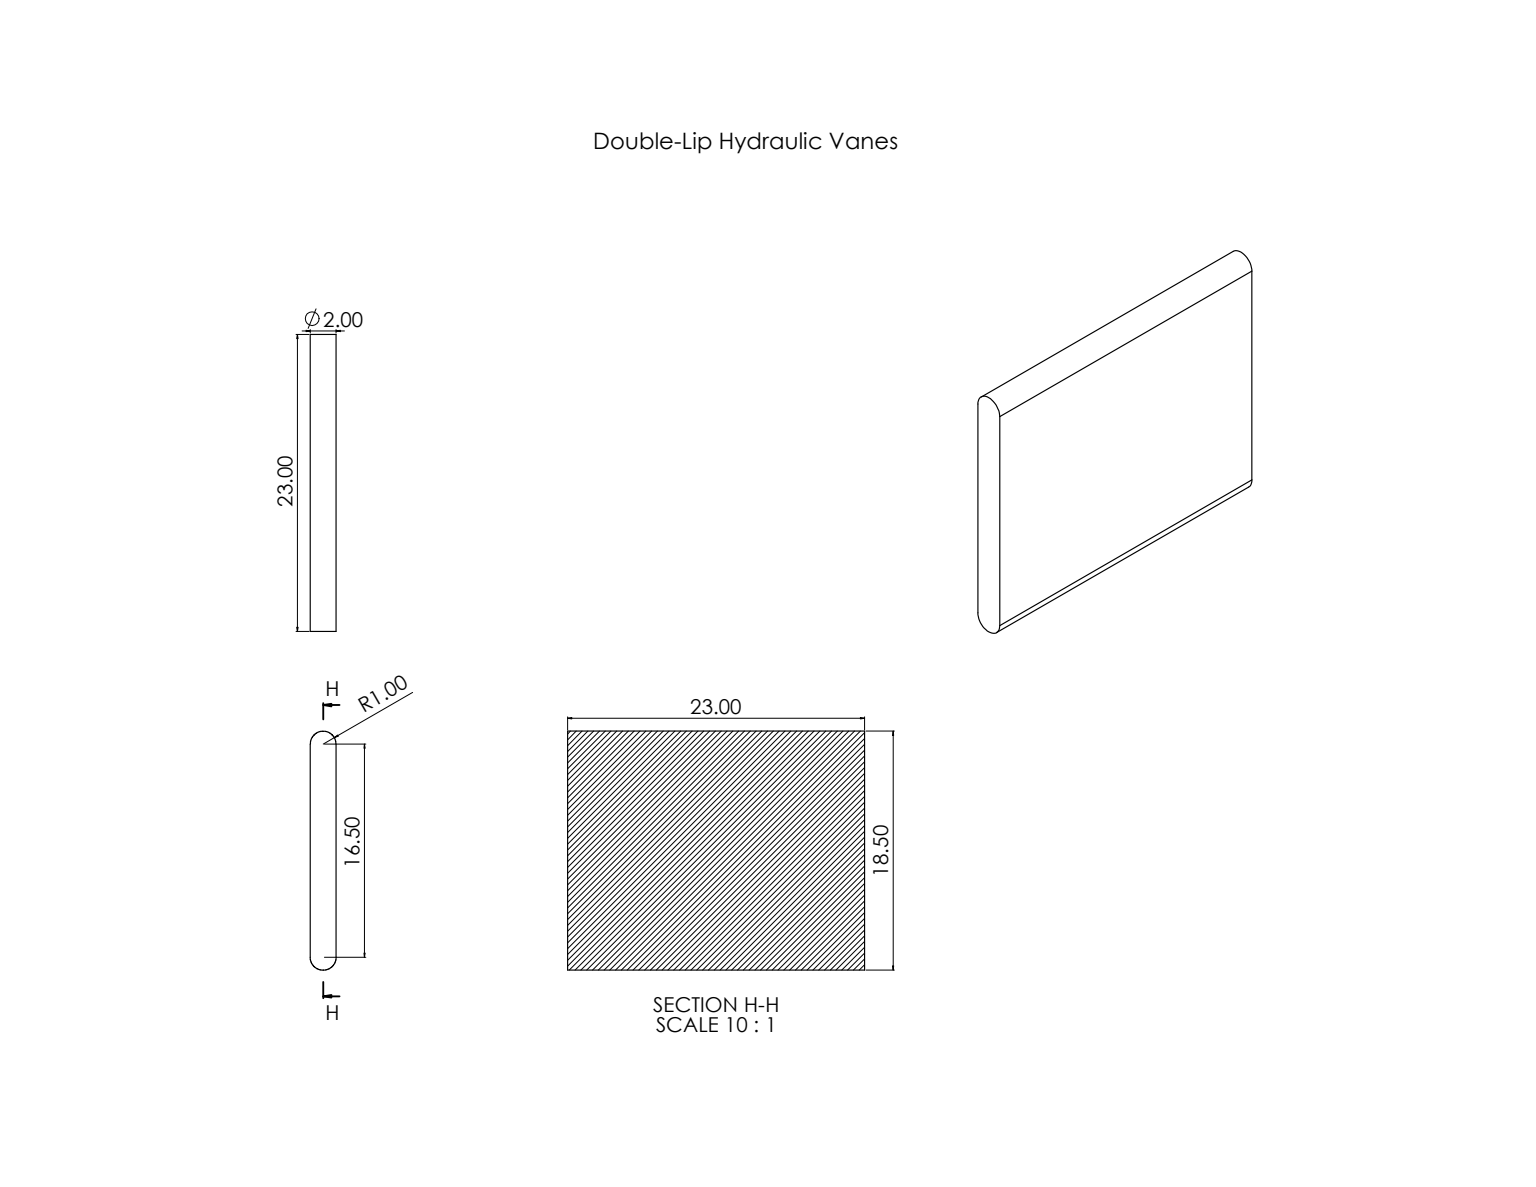
ISO-10303-21;
HEADER;
FILE_DESCRIPTION (('STEP AP214'),
    '1' );
FILE_NAME ('Double-Lip Hydraulic Vanes.step',
    '2026-10-18T20:16:25',
    ( '' ),
    ( '' ),
    'SwSTEP 2.0',
    'SolidWorks 2025',
    '' );
FILE_SCHEMA (( 'AUTOMOTIVE_DESIGN' ));
ENDSEC;

DATA;
#28=FACE_OUTER_BOUND ( 'NONE', #21455, .T. ) ;
#329=EDGE_LOOP ( 'NONE', ( #2074, #5797, #19024, #28874 ) ) ;
#819=AXIS2_PLACEMENT_3D ( 'NONE', #4409, #15801, #25484 ) ;
#861=CARTESIAN_POINT ( 'NONE',  ( 1.000000000000008438, 13.00000000000001421, 43.10779406592839536 ) ) ;
#935=PRODUCT_DEFINITION_FORMATION_WITH_SPECIFIED_SOURCE ( 'ANY', '', #4681, .NOT_KNOWN. ) ;
#968=EDGE_CURVE ( 'NONE', #15364, #12485, #28729, .T. ) ;
#978=ADVANCED_FACE ( 'NONE', ( #28 ), #7045, .T. ) ;
#1080=AXIS2_PLACEMENT_3D ( 'NONE', #18598, #6587, #14049 ) ;
#1081=CARTESIAN_POINT ( 'NONE',  ( 0.000000000000000000, 13.00000000000001421, 43.10779406592839536 ) ) ;
#1485=EDGE_LOOP ( 'NONE', ( #14703, #24943, #18019, #16923 ) ) ;
#1591=LINE ( 'NONE', #6710, #11635 ) ;
#1910=DIRECTION ( 'NONE',  ( 1.000000000000000000, 0.000000000000000000, 0.000000000000000000 ) ) ;
#2055=DIRECTION ( 'NONE',  ( 5.125319360840571077E-16, -1.000000000000000000, 0.000000000000000000 ) ) ;
#2074=ORIENTED_EDGE ( 'NONE', *, *, #968, .F. ) ;
#2224=CARTESIAN_POINT ( 'NONE',  ( -1.000000000000016875, 29.50000000000000000, 24.50000000000000000 ) ) ;
#2328=CIRCLE ( 'NONE', #819, 1.000000000000008438 ) ;
#2572=CIRCLE ( 'NONE', #1080, 1.000000000000008438 ) ;
#2682=DIRECTION ( 'NONE',  ( -0.000000000000000000, -0.000000000000000000, -1.000000000000000000 ) ) ;
#3020=VERTEX_POINT ( 'NONE', #17098 ) ;
#3096=VECTOR ( 'NONE', #3650, 1000.000000000000000 ) ;
#3213=DIRECTION ( 'NONE',  ( -0.000000000000000000, -0.000000000000000000, -1.000000000000000000 ) ) ;
#3406=( GEOMETRIC_REPRESENTATION_CONTEXT ( 3 ) GLOBAL_UNCERTAINTY_ASSIGNED_CONTEXT ( ( #6119 ) ) GLOBAL_UNIT_ASSIGNED_CONTEXT ( ( #26801, #5577, #24588 ) ) REPRESENTATION_CONTEXT ( 'NONE', 'WORKASPACE' ) );
#3624=DIRECTION ( 'NONE',  ( -0.000000000000000000, -0.000000000000000000, -1.000000000000000000 ) ) ;
#3650=DIRECTION ( 'NONE',  ( 5.125319360840571077E-16, -1.000000000000000000, 0.000000000000000000 ) ) ;
#3914=CIRCLE ( 'NONE', #20355, 1.000000000000008438 ) ;
#3950=ORIENTED_EDGE ( 'NONE', *, *, #25611, .F. ) ;
#3962=DIRECTION ( 'NONE',  ( -0.000000000000000000, -0.000000000000000000, -1.000000000000000000 ) ) ;
#4409=CARTESIAN_POINT ( 'NONE',  ( 0.000000000000000000, 13.00000000000001421, 24.50000000000000000 ) ) ;
#4468=EDGE_CURVE ( 'NONE', #12485, #24910, #2328, .T. ) ;
#4617=ADVANCED_FACE ( 'NONE', ( #7527 ), #19374, .T. ) ;
#4681=PRODUCT ( 'Double-Lip Hydraulic Vanes', 'Double-Lip Hydraulic Vanes', '', ( #28633 ) ) ;
#5176=DIRECTION ( 'NONE',  ( 1.000000000000000000, 0.000000000000000000, -0.000000000000000000 ) ) ;
#5178=VECTOR ( 'NONE', #18475, 1000.000000000000000 ) ;
#5306=ORIENTED_EDGE ( 'NONE', *, *, #15767, .F. ) ;
#5531=VERTEX_POINT ( 'NONE', #12235 ) ;
#5567=EDGE_CURVE ( 'NONE', #3020, #5531, #25324, .T. ) ;
#5577=( NAMED_UNIT ( * ) PLANE_ANGLE_UNIT ( ) SI_UNIT ( $, .RADIAN. ) );
#5797=ORIENTED_EDGE ( 'NONE', *, *, #15767, .T. ) ;
#5804=ADVANCED_FACE ( 'NONE', ( #24777 ), #21543, .T. ) ;
#6119=UNCERTAINTY_MEASURE_WITH_UNIT (LENGTH_MEASURE( 1.000000000000000082E-05 ), #26801, 'distance_accuracy_value', 'NONE');
#6266=CARTESIAN_POINT ( 'NONE',  ( -1.000000000000016875, 29.50000000000000000, 1.500000000000001332 ) ) ;
#6476=STYLED_ITEM('',(#30914),#12830);
#6537=ORIENTED_EDGE ( 'NONE', *, *, #4468, .T. ) ;
#6587=DIRECTION ( 'NONE',  ( 0.000000000000000000, 0.000000000000000000, 1.000000000000000000 ) ) ;
#6688=VECTOR ( 'NONE', #28371, 1000.000000000000000 ) ;
#6710=CARTESIAN_POINT ( 'NONE',  ( -1.000000000000008438, 13.00000000000001421, 43.10779406592839536 ) ) ;
#6888=ADVANCED_FACE ( 'NONE', ( #23732 ), #26237, .F. ) ;
#6895=CARTESIAN_POINT ( 'NONE',  ( -1.000000000000008438, 13.00000000000001421, 24.50000000000000000 ) ) ;
#7045=CYLINDRICAL_SURFACE ( 'NONE', #18847, 1.000000000000008438 ) ;
#7396=AXIS2_PLACEMENT_3D ( 'NONE', #9486, #28514, #21014 ) ;
#7421=ORIENTED_EDGE ( 'NONE', *, *, #27687, .F. ) ;
#7482=EDGE_CURVE ( 'NONE', #23974, #14320, #10448, .T. ) ;
#7499=ORIENTED_EDGE ( 'NONE', *, *, #27687, .T. ) ;
#7527=FACE_OUTER_BOUND ( 'NONE', #28761, .T. ) ;
#8090=AXIS2_PLACEMENT_3D ( 'NONE', #1081, #2682, #20107 ) ;
#8449=CARTESIAN_POINT ( 'NONE',  ( 1.000000000000000000, 29.50000000000000000, 24.50000000000000000 ) ) ;
#8861=ORIENTED_EDGE ( 'NONE', *, *, #28868, .F. ) ;
#8936=UNCERTAINTY_MEASURE_WITH_UNIT (LENGTH_MEASURE( 1.000000000000000082E-05 ), #12715, 'distance_accuracy_value', 'NONE');
#8960=CARTESIAN_POINT ( 'NONE',  ( 1.000000000000000000, 29.50000000000000000, 43.10779406592839536 ) ) ;
#9035=ORIENTED_EDGE ( 'NONE', *, *, #25213, .T. ) ;
#9486=CARTESIAN_POINT ( 'NONE',  ( 0.000000000000000000, 0.000000000000000000, 0.000000000000000000 ) ) ;
#9600=( NAMED_UNIT ( * ) SI_UNIT ( $, .STERADIAN. ) SOLID_ANGLE_UNIT ( ) );
#10319=DIRECTION ( 'NONE',  ( -5.125319360840571077E-16, 1.000000000000000000, 0.000000000000000000 ) ) ;
#10335=AXIS2_PLACEMENT_3D ( 'NONE', #16880, #28734, #5176 ) ;
#10394=APPLICATION_CONTEXT ( 'automotive_design' ) ;
#10411=ORIENTED_EDGE ( 'NONE', *, *, #14353, .F. ) ;
#10448=LINE ( 'NONE', #20114, #12090 ) ;
#10461=MECHANICAL_DESIGN_GEOMETRIC_PRESENTATION_REPRESENTATION('',(#6476),#22412);
#10877=VECTOR ( 'NONE', #2055, 1000.000000000000000 ) ;
#11065=DIRECTION ( 'NONE',  ( -5.125319360840571077E-16, 1.000000000000000000, 0.000000000000000000 ) ) ;
#11101=DIRECTION ( 'NONE',  ( -0.000000000000000000, -0.000000000000000000, -1.000000000000000000 ) ) ;
#11635=VECTOR ( 'NONE', #11101, 1000.000000000000000 ) ;
#12090=VECTOR ( 'NONE', #11065, 1000.000000000000000 ) ;
#12235=CARTESIAN_POINT ( 'NONE',  ( 1.000000000000008438, 13.00000000000001421, 1.500000000000001332 ) ) ;
#12485=VERTEX_POINT ( 'NONE', #27708 ) ;
#12521=FACE_OUTER_BOUND ( 'NONE', #329, .T. ) ;
#12677=DIRECTION ( 'NONE',  ( 1.000000000000000000, 5.125319360840571077E-16, -0.000000000000000000 ) ) ;
#12715=( LENGTH_UNIT ( ) NAMED_UNIT ( * ) SI_UNIT ( .MILLI., .METRE. ) );
#12830=MANIFOLD_SOLID_BREP ( 'Boss-Extrude4', #15814 ) ;
#13182=VECTOR ( 'NONE', #3624, 1000.000000000000000 ) ;
#13382=ORIENTED_EDGE ( 'NONE', *, *, #14434, .T. ) ;
#13933=LINE ( 'NONE', #8960, #5178 ) ;
#14049=DIRECTION ( 'NONE',  ( 1.000000000000000000, 0.000000000000000000, 0.000000000000000000 ) ) ;
#14320=VERTEX_POINT ( 'NONE', #6266 ) ;
#14353=EDGE_CURVE ( 'NONE', #24910, #5531, #17827, .T. ) ;
#14434=EDGE_CURVE ( 'NONE', #12485, #23974, #1591, .T. ) ;
#14493=VECTOR ( 'NONE', #22857, 1000.000000000000000 ) ;
#14665=PRODUCT_DEFINITION ( 'UNKNOWN', '', #935, #18249 ) ;
#14703=ORIENTED_EDGE ( 'NONE', *, *, #25213, .F. ) ;
#14842=CARTESIAN_POINT ( 'NONE',  ( -1.000000000000008438, 13.00000000000001421, 43.10779406592839536 ) ) ;
#14894=SHAPE_DEFINITION_REPRESENTATION ( #30827, #28257 ) ;
#15364=VERTEX_POINT ( 'NONE', #2224 ) ;
#15389=ORIENTED_EDGE ( 'NONE', *, *, #7482, .T. ) ;
#15446=EDGE_CURVE ( 'NONE', #22212, #3020, #13933, .T. ) ;
#15767=EDGE_CURVE ( 'NONE', #15364, #14320, #18854, .T. ) ;
#15801=DIRECTION ( 'NONE',  ( 0.000000000000000000, 0.000000000000000000, 1.000000000000000000 ) ) ;
#15814=CLOSED_SHELL ( 'NONE', ( #5804, #30028, #978, #17412, #4617, #6888 ) ) ;
#16100=AXIS2_PLACEMENT_3D ( 'NONE', #28286, #21401, #30765 ) ;
#16127=ORIENTED_EDGE ( 'NONE', *, *, #968, .T. ) ;
#16880=CARTESIAN_POINT ( 'NONE',  ( -4.163336342344337027E-14, 1.387778780781445676E-14, 24.50000000000000000 ) ) ;
#16923=ORIENTED_EDGE ( 'NONE', *, *, #15446, .F. ) ;
#17098=CARTESIAN_POINT ( 'NONE',  ( 1.000000000000000000, 29.50000000000000000, 1.500000000000001332 ) ) ;
#17412=ADVANCED_FACE ( 'NONE', ( #12521 ), #22170, .F. ) ;
#17553=DIRECTION ( 'NONE',  ( -1.000000000000000000, -5.125319360840571077E-16, 0.000000000000000000 ) ) ;
#17688=EDGE_LOOP ( 'NONE', ( #22391, #13382, #7421, #10411 ) ) ;
#17827=LINE ( 'NONE', #24985, #13182 ) ;
#17884=DIRECTION ( 'NONE',  ( 1.000000000000000000, 0.000000000000000000, 0.000000000000000000 ) ) ;
#18019=ORIENTED_EDGE ( 'NONE', *, *, #5567, .F. ) ;
#18156=CARTESIAN_POINT ( 'NONE',  ( 1.000000000000008438, 13.00000000000001421, 1.500000000000001332 ) ) ;
#18249=PRODUCT_DEFINITION_CONTEXT ( 'detailed design', #10394, 'design' ) ;
#18475=DIRECTION ( 'NONE',  ( -0.000000000000000000, -0.000000000000000000, -1.000000000000000000 ) ) ;
#18577=ORIENTED_EDGE ( 'NONE', *, *, #28868, .T. ) ;
#18598=CARTESIAN_POINT ( 'NONE',  ( -8.456776945386934585E-15, 29.50000000000000000, 24.50000000000000000 ) ) ;
#18606=DIRECTION ( 'NONE',  ( -0.000000000000000000, -0.000000000000000000, -1.000000000000000000 ) ) ;
#18847=AXIS2_PLACEMENT_3D ( 'NONE', #26392, #18606, #28118 ) ;
#18854=LINE ( 'NONE', #21158, #6688 ) ;
#19024=ORIENTED_EDGE ( 'NONE', *, *, #7482, .F. ) ;
#19374=PLANE ( 'NONE',  #10335 ) ;
#20107=DIRECTION ( 'NONE',  ( -1.000000000000000000, 0.000000000000000000, 0.000000000000000000 ) ) ;
#20114=CARTESIAN_POINT ( 'NONE',  ( -1.000000000000008438, 13.00000000000001421, 1.500000000000001332 ) ) ;
#20355=AXIS2_PLACEMENT_3D ( 'NONE', #22684, #3213, #17884 ) ;
#21014=DIRECTION ( 'NONE',  ( 1.000000000000000000, 0.000000000000000000, 0.000000000000000000 ) ) ;
#21158=CARTESIAN_POINT ( 'NONE',  ( -1.000000000000016875, 29.50000000000000000, 43.10779406592839536 ) ) ;
#21401=DIRECTION ( 'NONE',  ( 0.000000000000000000, 0.000000000000000000, 1.000000000000000000 ) ) ;
#21455=EDGE_LOOP ( 'NONE', ( #3950, #26929, #8861, #5306 ) ) ;
#21543=CYLINDRICAL_SURFACE ( 'NONE', #8090, 1.000000000000008438 ) ;
#21637=SHAPE_REPRESENTATION_RELATIONSHIP ( 'NONE' , 'NONE' ,  #28257, #30671 ) ;
#21817=CARTESIAN_POINT ( 'NONE',  ( 1.000000000000008438, 13.00000000000001421, 24.50000000000000000 ) ) ;
#22139=ORIENTED_EDGE ( 'NONE', *, *, #5567, .T. ) ;
#22170=PLANE ( 'NONE',  #27186 ) ;
#22212=VERTEX_POINT ( 'NONE', #8449 ) ;
#22391=ORIENTED_EDGE ( 'NONE', *, *, #4468, .F. ) ;
#22412=( GEOMETRIC_REPRESENTATION_CONTEXT ( 3 ) GLOBAL_UNCERTAINTY_ASSIGNED_CONTEXT ( ( #8936 ) ) GLOBAL_UNIT_ASSIGNED_CONTEXT ( ( #12715, #29240, #9600 ) ) REPRESENTATION_CONTEXT ( 'NONE', 'WORKASPACE' ) );
#22684=CARTESIAN_POINT ( 'NONE',  ( -8.456776945386934585E-15, 29.50000000000000000, 1.500000000000001332 ) ) ;
#22795=AXIS2_PLACEMENT_3D ( 'NONE', #861, #17553, #24713 ) ;
#22857=DIRECTION ( 'NONE',  ( -5.125319360840571077E-16, 1.000000000000000000, 0.000000000000000000 ) ) ;
#23571=EDGE_LOOP ( 'NONE', ( #7499, #15389, #18577, #22139 ) ) ;
#23732=FACE_OUTER_BOUND ( 'NONE', #23571, .T. ) ;
#23974=VERTEX_POINT ( 'NONE', #29987 ) ;
#24471=ORIENTED_EDGE ( 'NONE', *, *, #25611, .T. ) ;
#24588=( NAMED_UNIT ( * ) SI_UNIT ( $, .STERADIAN. ) SOLID_ANGLE_UNIT ( ) );
#24713=DIRECTION ( 'NONE',  ( 5.125319360840571077E-16, -1.000000000000000000, 0.000000000000000000 ) ) ;
#24777=FACE_OUTER_BOUND ( 'NONE', #17688, .T. ) ;
#24910=VERTEX_POINT ( 'NONE', #21817 ) ;
#24943=ORIENTED_EDGE ( 'NONE', *, *, #14353, .T. ) ;
#24985=CARTESIAN_POINT ( 'NONE',  ( 1.000000000000008438, 13.00000000000001421, 43.10779406592839536 ) ) ;
#25047=LINE ( 'NONE', #25193, #14493 ) ;
#25193=CARTESIAN_POINT ( 'NONE',  ( 1.000000000000008438, 13.00000000000001421, 24.50000000000000000 ) ) ;
#25213=EDGE_CURVE ( 'NONE', #24910, #22212, #25047, .T. ) ;
#25324=LINE ( 'NONE', #18156, #3096 ) ;
#25484=DIRECTION ( 'NONE',  ( 1.000000000000000000, 0.000000000000000000, 0.000000000000000000 ) ) ;
#25611=EDGE_CURVE ( 'NONE', #22212, #15364, #2572, .T. ) ;
#26237=PLANE ( 'NONE',  #16100 ) ;
#26392=CARTESIAN_POINT ( 'NONE',  ( -8.456776945386934585E-15, 29.50000000000000000, 43.10779406592839536 ) ) ;
#26560=CIRCLE ( 'NONE', #30534, 1.000000000000008438 ) ;
#26614=FACE_OUTER_BOUND ( 'NONE', #1485, .T. ) ;
#26801=( LENGTH_UNIT ( ) NAMED_UNIT ( * ) SI_UNIT ( .MILLI., .METRE. ) );
#26929=ORIENTED_EDGE ( 'NONE', *, *, #15446, .T. ) ;
#27186=AXIS2_PLACEMENT_3D ( 'NONE', #14842, #12677, #10319 ) ;
#27687=EDGE_CURVE ( 'NONE', #5531, #23974, #26560, .T. ) ;
#27708=CARTESIAN_POINT ( 'NONE',  ( -1.000000000000008438, 13.00000000000001421, 24.50000000000000000 ) ) ;
#27821=CARTESIAN_POINT ( 'NONE',  ( 0.000000000000000000, 13.00000000000001421, 1.500000000000001332 ) ) ;
#28111=APPLICATION_CONTEXT ( 'automotive_design' ) ;
#28118=DIRECTION ( 'NONE',  ( -1.000000000000000000, 0.000000000000000000, 0.000000000000000000 ) ) ;
#28257=SHAPE_REPRESENTATION ( 'Double-Lip Hydraulic Vanes', ( #7396 ), #3406 ) ;
#28286=CARTESIAN_POINT ( 'NONE',  ( -4.163336342344337027E-14, 1.387778780781445676E-14, 1.500000000000000000 ) ) ;
#28371=DIRECTION ( 'NONE',  ( -0.000000000000000000, -0.000000000000000000, -1.000000000000000000 ) ) ;
#28514=DIRECTION ( 'NONE',  ( 0.000000000000000000, 0.000000000000000000, 1.000000000000000000 ) ) ;
#28633=PRODUCT_CONTEXT ( 'NONE', #28111, 'mechanical' ) ;
#28729=LINE ( 'NONE', #6895, #10877 ) ;
#28734=DIRECTION ( 'NONE',  ( 0.000000000000000000, 0.000000000000000000, 1.000000000000000000 ) ) ;
#28761=EDGE_LOOP ( 'NONE', ( #16127, #6537, #9035, #24471 ) ) ;
#28868=EDGE_CURVE ( 'NONE', #14320, #3020, #3914, .T. ) ;
#28874=ORIENTED_EDGE ( 'NONE', *, *, #14434, .F. ) ;
#29240=( NAMED_UNIT ( * ) PLANE_ANGLE_UNIT ( ) SI_UNIT ( $, .RADIAN. ) );
#29256=PLANE ( 'NONE',  #22795 ) ;
#29987=CARTESIAN_POINT ( 'NONE',  ( -1.000000000000008438, 13.00000000000001421, 1.500000000000001332 ) ) ;
#30028=ADVANCED_FACE ( 'NONE', ( #26614 ), #29256, .F. ) ;
#30534=AXIS2_PLACEMENT_3D ( 'NONE', #27821, #3962, #1910 ) ;
#30671=ADVANCED_BREP_SHAPE_REPRESENTATION ( '', ( #12830, #7396 ), #3406 ) ;
#30765=DIRECTION ( 'NONE',  ( 1.000000000000000000, 0.000000000000000000, -0.000000000000000000 ) ) ;
#30827=PRODUCT_DEFINITION_SHAPE ( 'NONE', 'NONE',  #14665 ) ;
#30908=COLOUR_RGB('Off White',0.89,0.88,0.83);
#30909=FILL_AREA_STYLE_COLOUR('',#30908);
#30910=FILL_AREA_STYLE('',(#30909));
#30911=SURFACE_STYLE_FILL_AREA(#30910);
#30912=SURFACE_SIDE_STYLE('',(#30911));
#30913=SURFACE_STYLE_USAGE(.BOTH.,#30912);
#30914=PRESENTATION_STYLE_ASSIGNMENT((#30913));
ENDSEC;
END-ISO-10303-21;
